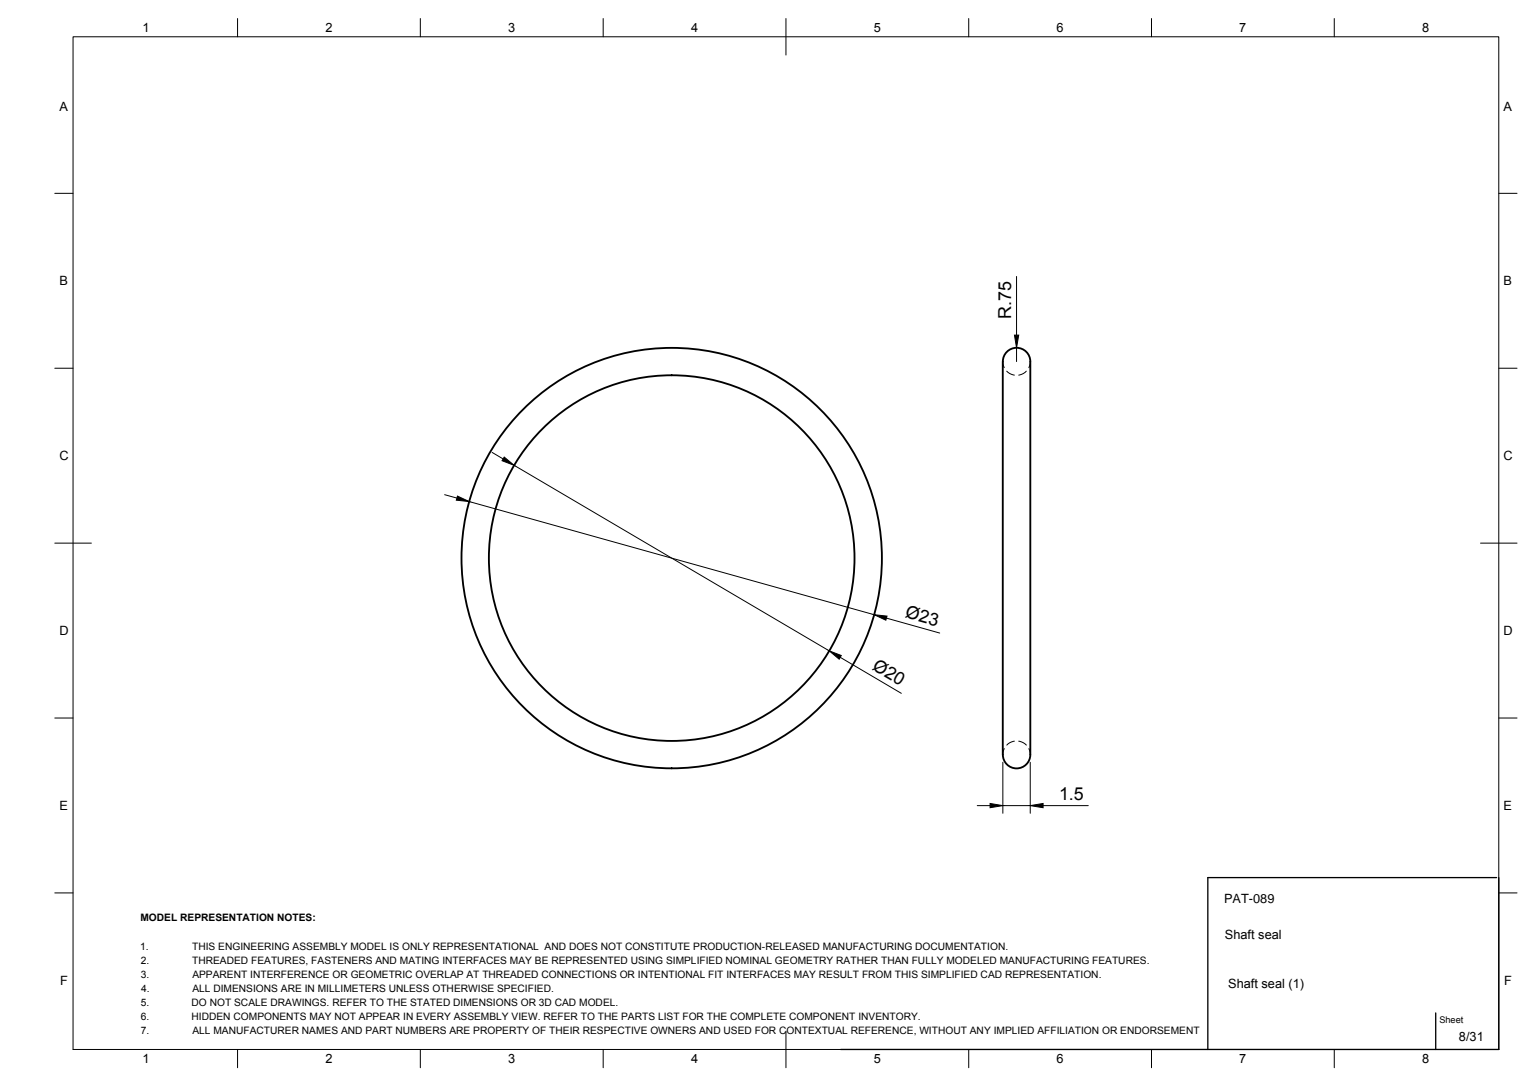
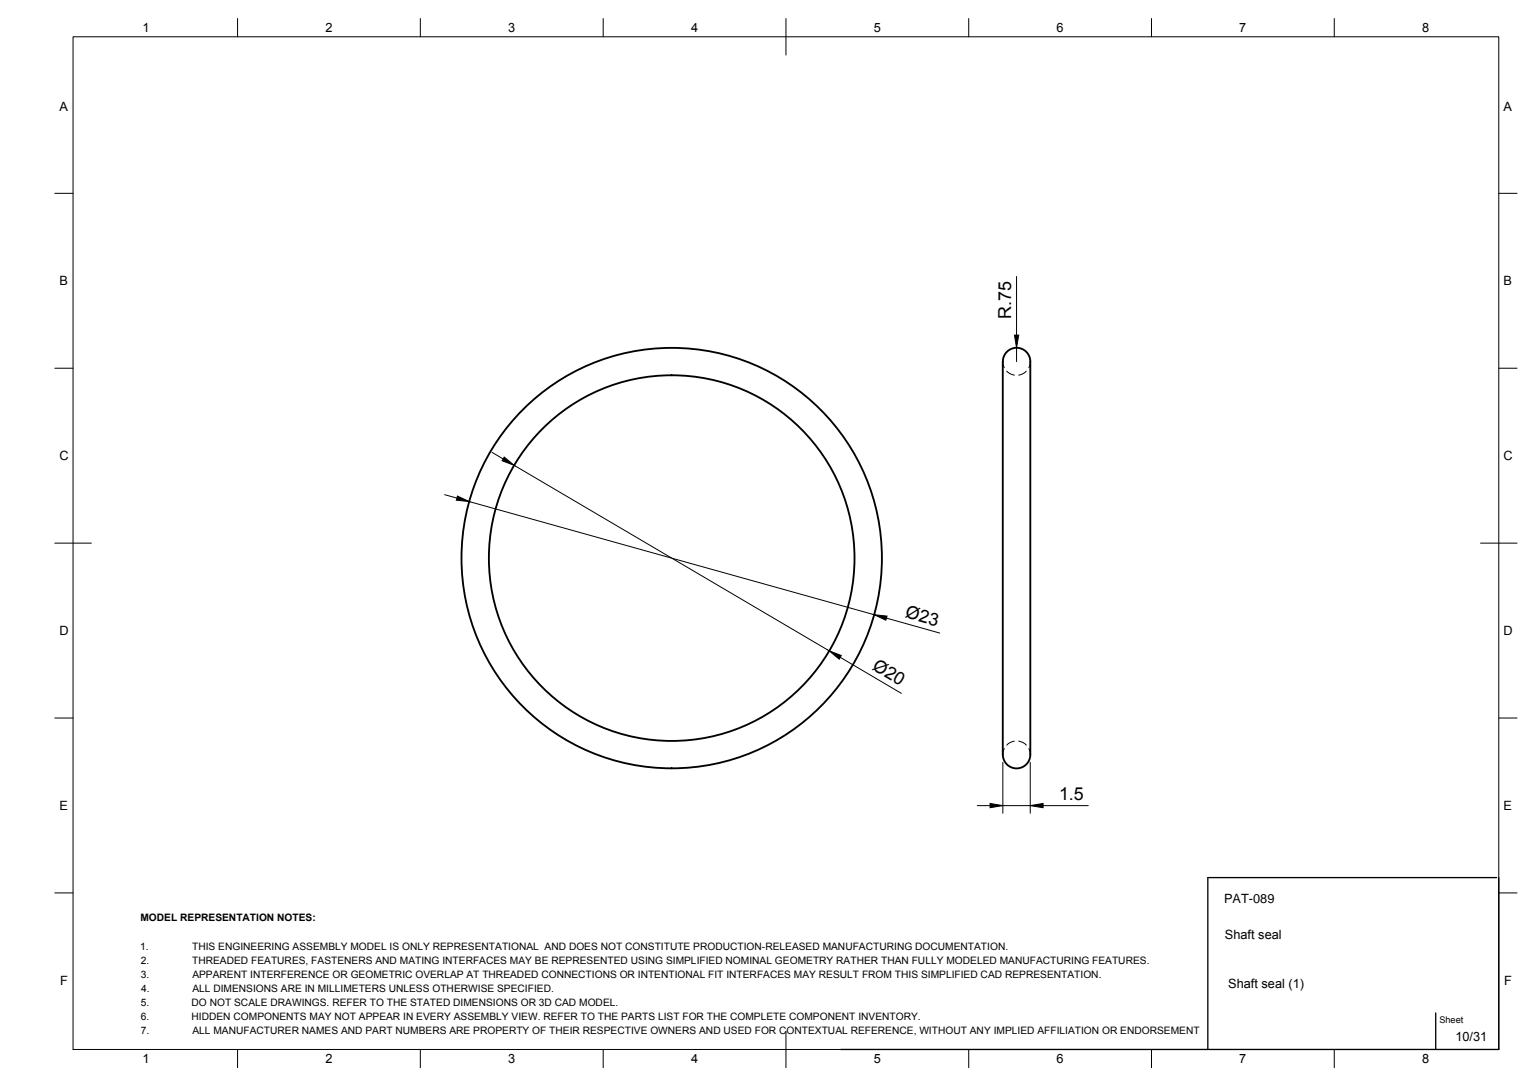
ISO-10303-21;
HEADER;
/* Generated by software containing ST-Developer
 * from STEP Tools, Inc. (www.steptools.com) 
 */

FILE_DESCRIPTION(
/* description */ ('Rotary union on bearing shaft'),
/* implementation_level */ '2;1');

FILE_NAME(
/* name */ 'Shaft seal.step',
/* time_stamp */ '2026-10-28T03:24:01-07:00',
/* author */ (''),
/* organization */ (''),
/* preprocessor_version */ 'ST-DEVELOPER v20.2',
/* originating_system */ 'Autodesk Translation Framework v15.17.0.0',
/* authorisation */ '');

FILE_SCHEMA (('AUTOMOTIVE_DESIGN { 1 0 10303 214 3 1 1 }'));
ENDSEC;

DATA;
#10=MECHANICAL_DESIGN_GEOMETRIC_PRESENTATION_REPRESENTATION('',(#316),#9448);
#221=TOROIDAL_SURFACE('',#5323,1.075,0.075);
#262=SHAPE_REPRESENTATION_RELATIONSHIP('SRR','None',#9562,#289);
#289=ADVANCED_BREP_SHAPE_REPRESENTATION('',(#351),#9422);
#316=STYLED_ITEM('',(#9785),#351);
#351=MANIFOLD_SOLID_BREP('Body1',#4871);
#717=FACE_OUTER_BOUND('',#1050,.T.);
#1050=EDGE_LOOP('',(#3521,#3522,#3523,#3524));
#2053=CIRCLE('',#5324,0.075);
#2054=CIRCLE('',#5325,1.);
#2337=VERTEX_POINT('',#7743);
#2788=EDGE_CURVE('',#2337,#2337,#2053,.T.);
#2789=EDGE_CURVE('',#2337,#2337,#2054,.T.);
#3521=ORIENTED_EDGE('',*,*,#2788,.F.);
#3522=ORIENTED_EDGE('',*,*,#2789,.T.);
#3523=ORIENTED_EDGE('',*,*,#2788,.T.);
#3524=ORIENTED_EDGE('',*,*,#2789,.F.);
#4630=ADVANCED_FACE('',(#717),#221,.T.);
#4871=CLOSED_SHELL('',(#4630));
#5322=AXIS2_PLACEMENT_3D('',#7741,#6135,#6136);
#5323=AXIS2_PLACEMENT_3D('',#7742,#6137,#6138);
#5324=AXIS2_PLACEMENT_3D('',#7744,#6139,#6140);
#5325=AXIS2_PLACEMENT_3D('',#7745,#6141,#6142);
#6135=DIRECTION('axis',(0.,0.,1.));
#6136=DIRECTION('refdir',(1.,0.,0.));
#6137=DIRECTION('center_axis',(0.,-1.,0.));
#6138=DIRECTION('ref_axis',(0.,0.,-1.));
#6139=DIRECTION('center_axis',(-1.,0.,-1.22464679914735E-16));
#6140=DIRECTION('ref_axis',(-1.22464679914735E-16,0.,1.));
#6141=DIRECTION('center_axis',(0.,1.,0.));
#6142=DIRECTION('ref_axis',(0.,0.,-1.));
#7741=CARTESIAN_POINT('',(0.,0.,0.));
#7742=CARTESIAN_POINT('Origin',(0.,2.05,4.5));
#7743=CARTESIAN_POINT('',(-1.22464679914735E-16,2.05,5.5));
#7744=CARTESIAN_POINT('Origin',(-1.3164953090834E-16,2.05,5.575));
#7745=CARTESIAN_POINT('Origin',(0.,2.05,4.5));
#9390=UNCERTAINTY_MEASURE_WITH_UNIT(LENGTH_MEASURE(0.001),#9449,
'DISTANCE_ACCURACY_VALUE',
'Maximum model space distance between geometric entities at asserted c
onnectivities');
#9416=UNCERTAINTY_MEASURE_WITH_UNIT(LENGTH_MEASURE(0.001),#9449,
'DISTANCE_ACCURACY_VALUE',
'Maximum model space distance between geometric entities at asserted c
onnectivities');
#9422=(
GEOMETRIC_REPRESENTATION_CONTEXT(3)
GLOBAL_UNCERTAINTY_ASSIGNED_CONTEXT((#9390))
GLOBAL_UNIT_ASSIGNED_CONTEXT((#9449,#9451,#9452))
REPRESENTATION_CONTEXT('','3D')
);
#9448=(
GEOMETRIC_REPRESENTATION_CONTEXT(3)
GLOBAL_UNCERTAINTY_ASSIGNED_CONTEXT((#9416))
GLOBAL_UNIT_ASSIGNED_CONTEXT((#9449,#9451,#9452))
REPRESENTATION_CONTEXT('','3D')
);
#9449=(
LENGTH_UNIT()
NAMED_UNIT(*)
SI_UNIT(.CENTI.,.METRE.)
);
#9451=(
NAMED_UNIT(*)
PLANE_ANGLE_UNIT()
SI_UNIT($,.RADIAN.)
);
#9452=(
NAMED_UNIT(*)
SI_UNIT($,.STERADIAN.)
SOLID_ANGLE_UNIT()
);
#9458=SHAPE_DEFINITION_REPRESENTATION(#9489,#9562);
#9489=PRODUCT_DEFINITION_SHAPE('',$,#9594);
#9562=SHAPE_REPRESENTATION('',(#5322),#9422);
#9588=PRODUCT_DEFINITION_CONTEXT('part definition',#9683,'design');
#9594=PRODUCT_DEFINITION('Shaft seal','Shaft seal',#9625,#9588);
#9625=PRODUCT_DEFINITION_FORMATION('',$,#9690);
#9683=APPLICATION_CONTEXT(
'Core Data for Automotive Mechanical Design Process');
#9684=PRODUCT_CONTEXT('part definition',#9683,'mechanical');
#9690=PRODUCT('Shaft seal','Shaft seal','Shaft seal',(#9684));
#9779=COLOUR_RGB('Black',0.12,0.14,0.17);
#9780=FILL_AREA_STYLE_COLOUR('',#9779);
#9781=FILL_AREA_STYLE('',(#9780));
#9782=SURFACE_STYLE_FILL_AREA(#9781);
#9783=SURFACE_SIDE_STYLE('',(#9782));
#9784=SURFACE_STYLE_USAGE(.BOTH.,#9783);
#9785=PRESENTATION_STYLE_ASSIGNMENT((#9784));
ENDSEC;
END-ISO-10303-21;
